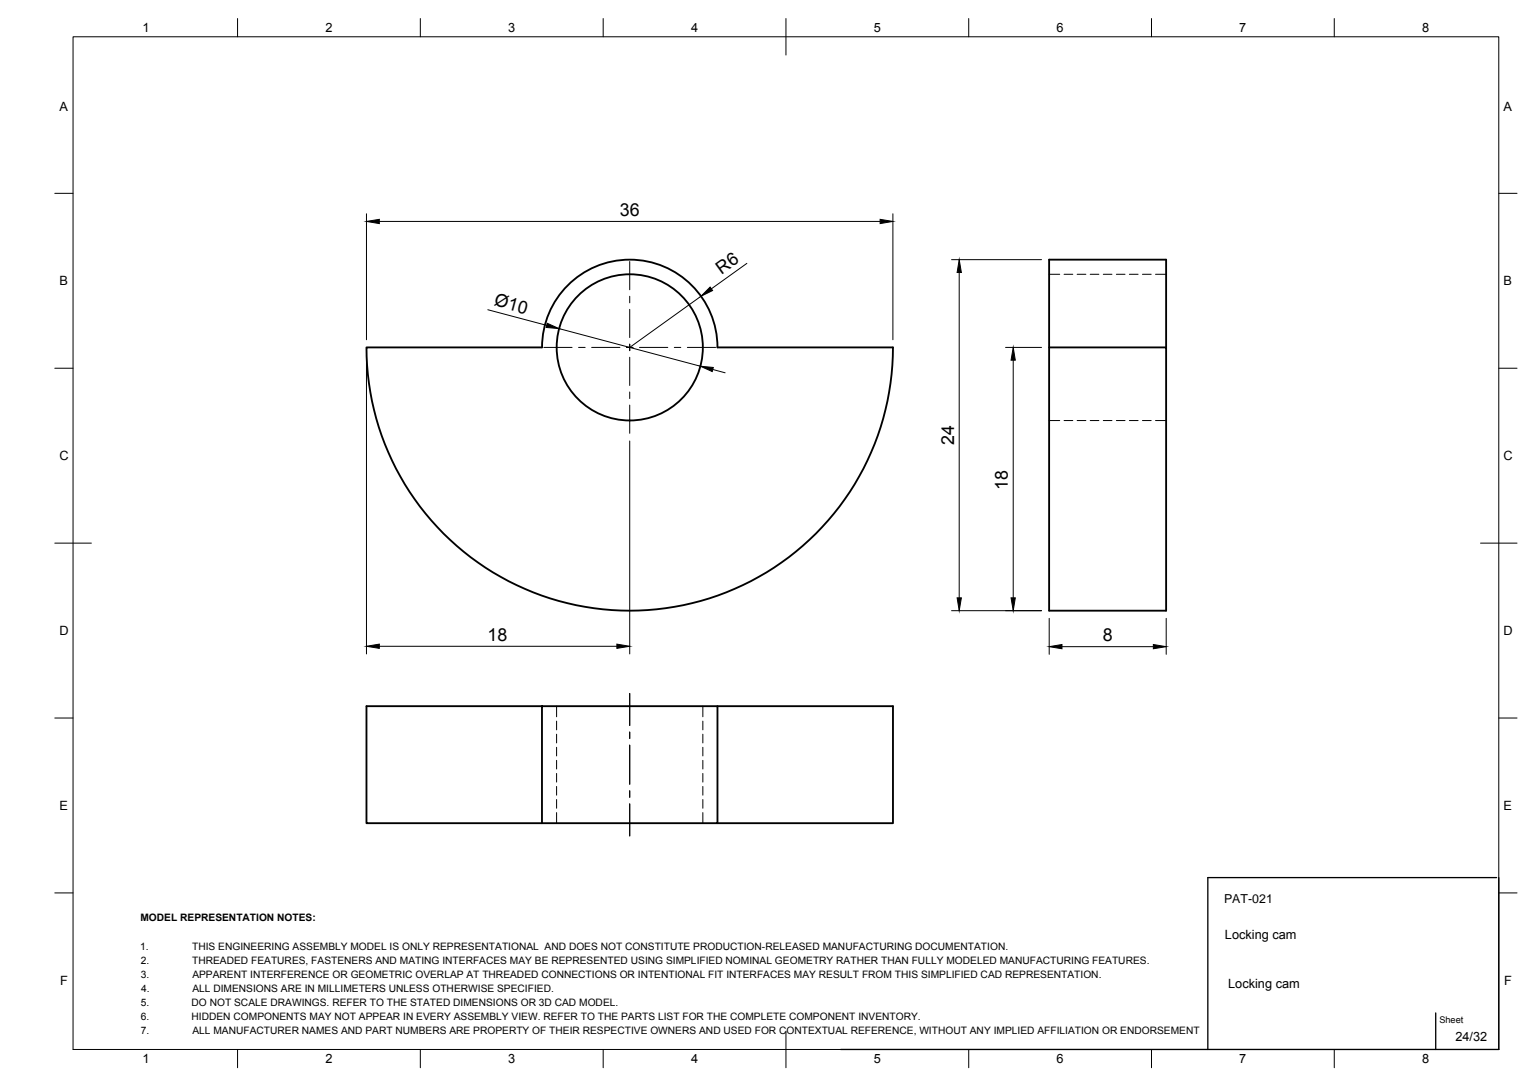
ISO-10303-21;
HEADER;
/* Generated by software containing ST-Developer
 * from STEP Tools, Inc. (www.steptools.com) 
 */

FILE_DESCRIPTION(
/* description */ ('Chain-less indexing wheel (Geneva) drive'),
/* implementation_level */ '2;1');

FILE_NAME(
/* name */ 'Locking cam.step',
/* time_stamp */ '2026-10-28T03:25:22-07:00',
/* author */ (''),
/* organization */ (''),
/* preprocessor_version */ 'ST-DEVELOPER v20.2',
/* originating_system */ 'Autodesk Translation Framework v15.17.0.0',
/* authorisation */ '');

FILE_SCHEMA (('AUTOMOTIVE_DESIGN { 1 0 10303 214 3 1 1 }'));
ENDSEC;

DATA;
#10=MECHANICAL_DESIGN_GEOMETRIC_PRESENTATION_REPRESENTATION('',(#327),#10957);
#269=SHAPE_REPRESENTATION_RELATIONSHIP('SRR','None',#11084,#294);
#294=ADVANCED_BREP_SHAPE_REPRESENTATION('',(#359),#10947);
#327=STYLED_ITEM('',(#11280),#359);
#359=MANIFOLD_SOLID_BREP('Body1',#5724);
#447=FACE_BOUND('',#1284,.T.);
#448=FACE_BOUND('',#1289,.T.);
#579=PLANE('',#6491);
#580=PLANE('',#6493);
#581=PLANE('',#6494);
#582=PLANE('',#6497);
#868=FACE_OUTER_BOUND('',#1281,.T.);
#869=FACE_OUTER_BOUND('',#1282,.T.);
#870=FACE_OUTER_BOUND('',#1283,.T.);
#871=FACE_OUTER_BOUND('',#1285,.T.);
#872=FACE_OUTER_BOUND('',#1286,.T.);
#873=FACE_OUTER_BOUND('',#1287,.T.);
#874=FACE_OUTER_BOUND('',#1288,.T.);
#1281=EDGE_LOOP('',(#4677,#4678,#4679,#4680));
#1282=EDGE_LOOP('',(#4681,#4682,#4683,#4684));
#1283=EDGE_LOOP('',(#4685,#4686,#4687,#4688));
#1284=EDGE_LOOP('',(#4689));
#1285=EDGE_LOOP('',(#4690,#4691,#4692,#4693));
#1286=EDGE_LOOP('',(#4694,#4695,#4696,#4697));
#1287=EDGE_LOOP('',(#4698,#4699,#4700,#4701));
#1288=EDGE_LOOP('',(#4702,#4703,#4704,#4705));
#1289=EDGE_LOOP('',(#4706));
#1625=LINE('',#10145,#1999);
#1626=LINE('',#10150,#2000);
#1627=LINE('',#10154,#2001);
#1628=LINE('',#10158,#2002);
#1629=LINE('',#10161,#2003);
#1630=LINE('',#10164,#2004);
#1631=LINE('',#10165,#2005);
#1632=LINE('',#10168,#2006);
#1633=LINE('',#10169,#2007);
#1999=VECTOR('',#7905,0.5);
#2000=VECTOR('',#7910,1.);
#2001=VECTOR('',#7913,1.);
#2002=VECTOR('',#7918,1.);
#2003=VECTOR('',#7921,1.);
#2004=VECTOR('',#7924,1.);
#2005=VECTOR('',#7925,1.);
#2006=VECTOR('',#7928,1.);
#2007=VECTOR('',#7929,1.);
#2404=CIRCLE('',#6486,0.5);
#2405=CIRCLE('',#6487,0.5);
#2406=CIRCLE('',#6489,0.6);
#2407=CIRCLE('',#6490,0.6);
#2408=CIRCLE('',#6492,1.8);
#2409=CIRCLE('',#6496,1.8);
#2812=VERTEX_POINT('',#10142);
#2813=VERTEX_POINT('',#10144);
#2814=VERTEX_POINT('',#10148);
#2815=VERTEX_POINT('',#10149);
#2816=VERTEX_POINT('',#10151);
#2817=VERTEX_POINT('',#10153);
#2818=VERTEX_POINT('',#10157);
#2819=VERTEX_POINT('',#10159);
#2820=VERTEX_POINT('',#10163);
#2821=VERTEX_POINT('',#10167);
#3464=EDGE_CURVE('',#2812,#2812,#2404,.T.);
#3465=EDGE_CURVE('',#2812,#2813,#1625,.T.);
#3466=EDGE_CURVE('',#2813,#2813,#2405,.T.);
#3467=EDGE_CURVE('',#2814,#2815,#1626,.T.);
#3468=EDGE_CURVE('',#2816,#2814,#2406,.T.);
#3469=EDGE_CURVE('',#2817,#2816,#1627,.T.);
#3470=EDGE_CURVE('',#2817,#2815,#2407,.T.);
#3471=EDGE_CURVE('',#2817,#2818,#1628,.T.);
#3472=EDGE_CURVE('',#2819,#2818,#2408,.T.);
#3473=EDGE_CURVE('',#2819,#2815,#1629,.T.);
#3474=EDGE_CURVE('',#2820,#2816,#1630,.T.);
#3475=EDGE_CURVE('',#2818,#2820,#1631,.T.);
#3476=EDGE_CURVE('',#2821,#2819,#1632,.T.);
#3477=EDGE_CURVE('',#2814,#2821,#1633,.T.);
#3478=EDGE_CURVE('',#2821,#2820,#2409,.T.);
#4677=ORIENTED_EDGE('',*,*,#3464,.F.);
#4678=ORIENTED_EDGE('',*,*,#3465,.T.);
#4679=ORIENTED_EDGE('',*,*,#3466,.F.);
#4680=ORIENTED_EDGE('',*,*,#3465,.F.);
#4681=ORIENTED_EDGE('',*,*,#3467,.F.);
#4682=ORIENTED_EDGE('',*,*,#3468,.F.);
#4683=ORIENTED_EDGE('',*,*,#3469,.F.);
#4684=ORIENTED_EDGE('',*,*,#3470,.T.);
#4685=ORIENTED_EDGE('',*,*,#3471,.T.);
#4686=ORIENTED_EDGE('',*,*,#3472,.F.);
#4687=ORIENTED_EDGE('',*,*,#3473,.T.);
#4688=ORIENTED_EDGE('',*,*,#3470,.F.);
#4689=ORIENTED_EDGE('',*,*,#3464,.T.);
#4690=ORIENTED_EDGE('',*,*,#3469,.T.);
#4691=ORIENTED_EDGE('',*,*,#3474,.F.);
#4692=ORIENTED_EDGE('',*,*,#3475,.F.);
#4693=ORIENTED_EDGE('',*,*,#3471,.F.);
#4694=ORIENTED_EDGE('',*,*,#3467,.T.);
#4695=ORIENTED_EDGE('',*,*,#3473,.F.);
#4696=ORIENTED_EDGE('',*,*,#3476,.F.);
#4697=ORIENTED_EDGE('',*,*,#3477,.F.);
#4698=ORIENTED_EDGE('',*,*,#3476,.T.);
#4699=ORIENTED_EDGE('',*,*,#3472,.T.);
#4700=ORIENTED_EDGE('',*,*,#3475,.T.);
#4701=ORIENTED_EDGE('',*,*,#3478,.F.);
#4702=ORIENTED_EDGE('',*,*,#3477,.T.);
#4703=ORIENTED_EDGE('',*,*,#3478,.T.);
#4704=ORIENTED_EDGE('',*,*,#3474,.T.);
#4705=ORIENTED_EDGE('',*,*,#3468,.T.);
#4706=ORIENTED_EDGE('',*,*,#3466,.T.);
#5326=CYLINDRICAL_SURFACE('',#6485,0.5);
#5327=CYLINDRICAL_SURFACE('',#6488,0.6);
#5328=CYLINDRICAL_SURFACE('',#6495,1.8);
#5582=ADVANCED_FACE('',(#868),#5326,.F.);
#5583=ADVANCED_FACE('',(#869),#5327,.T.);
#5584=ADVANCED_FACE('',(#870,#447),#579,.F.);
#5585=ADVANCED_FACE('',(#871),#580,.F.);
#5586=ADVANCED_FACE('',(#872),#581,.F.);
#5587=ADVANCED_FACE('',(#873),#5328,.T.);
#5588=ADVANCED_FACE('',(#874,#448),#582,.T.);
#5724=CLOSED_SHELL('',(#5582,#5583,#5584,#5585,#5586,#5587,#5588));
#6484=AXIS2_PLACEMENT_3D('',#10140,#7899,#7900);
#6485=AXIS2_PLACEMENT_3D('',#10141,#7901,#7902);
#6486=AXIS2_PLACEMENT_3D('',#10143,#7903,#7904);
#6487=AXIS2_PLACEMENT_3D('',#10146,#7906,#7907);
#6488=AXIS2_PLACEMENT_3D('',#10147,#7908,#7909);
#6489=AXIS2_PLACEMENT_3D('',#10152,#7911,#7912);
#6490=AXIS2_PLACEMENT_3D('',#10155,#7914,#7915);
#6491=AXIS2_PLACEMENT_3D('',#10156,#7916,#7917);
#6492=AXIS2_PLACEMENT_3D('',#10160,#7919,#7920);
#6493=AXIS2_PLACEMENT_3D('',#10162,#7922,#7923);
#6494=AXIS2_PLACEMENT_3D('',#10166,#7926,#7927);
#6495=AXIS2_PLACEMENT_3D('',#10170,#7930,#7931);
#6496=AXIS2_PLACEMENT_3D('',#10171,#7932,#7933);
#6497=AXIS2_PLACEMENT_3D('',#10172,#7934,#7935);
#7899=DIRECTION('axis',(0.,0.,1.));
#7900=DIRECTION('refdir',(1.,0.,0.));
#7901=DIRECTION('center_axis',(0.,0.,1.));
#7902=DIRECTION('ref_axis',(1.,0.,0.));
#7903=DIRECTION('center_axis',(0.,0.,1.));
#7904=DIRECTION('ref_axis',(1.,0.,0.));
#7905=DIRECTION('',(0.,0.,1.));
#7906=DIRECTION('center_axis',(0.,0.,-1.));
#7907=DIRECTION('ref_axis',(1.,0.,0.));
#7908=DIRECTION('center_axis',(0.,0.,1.));
#7909=DIRECTION('ref_axis',(1.,0.,0.));
#7910=DIRECTION('',(0.,0.,-1.));
#7911=DIRECTION('center_axis',(0.,0.,1.));
#7912=DIRECTION('ref_axis',(1.,0.,0.));
#7913=DIRECTION('',(0.,0.,1.));
#7914=DIRECTION('center_axis',(0.,0.,1.));
#7915=DIRECTION('ref_axis',(1.,0.,0.));
#7916=DIRECTION('center_axis',(0.,0.,1.));
#7917=DIRECTION('ref_axis',(1.,0.,0.));
#7918=DIRECTION('',(0.,-1.,0.));
#7919=DIRECTION('center_axis',(0.,0.,1.));
#7920=DIRECTION('ref_axis',(1.,0.,0.));
#7921=DIRECTION('',(0.,-1.,0.));
#7922=DIRECTION('center_axis',(-1.,0.,0.));
#7923=DIRECTION('ref_axis',(0.,-1.,0.));
#7924=DIRECTION('',(0.,1.,0.));
#7925=DIRECTION('',(0.,0.,1.));
#7926=DIRECTION('center_axis',(-1.,0.,0.));
#7927=DIRECTION('ref_axis',(0.,-1.,0.));
#7928=DIRECTION('',(0.,0.,-1.));
#7929=DIRECTION('',(0.,1.,0.));
#7930=DIRECTION('center_axis',(0.,0.,1.));
#7931=DIRECTION('ref_axis',(-1.,1.22464679914735E-16,0.));
#7932=DIRECTION('center_axis',(0.,0.,1.));
#7933=DIRECTION('ref_axis',(1.,0.,0.));
#7934=DIRECTION('center_axis',(0.,0.,1.));
#7935=DIRECTION('ref_axis',(1.,0.,0.));
#10140=CARTESIAN_POINT('',(0.,0.,0.));
#10141=CARTESIAN_POINT('Origin',(0.,0.,5.9));
#10142=CARTESIAN_POINT('',(-0.5,-6.12323399573677E-17,6.));
#10143=CARTESIAN_POINT('Origin',(0.,0.,6.));
#10144=CARTESIAN_POINT('',(-0.5,6.12323399573677E-17,6.8));
#10145=CARTESIAN_POINT('',(-0.5,-6.12323399573677E-17,5.9));
#10146=CARTESIAN_POINT('Origin',(0.,0.,6.8));
#10147=CARTESIAN_POINT('Origin',(0.,0.,6.));
#10148=CARTESIAN_POINT('',(0.,0.6,6.8));
#10149=CARTESIAN_POINT('',(0.,0.6,6.));
#10150=CARTESIAN_POINT('',(0.,0.6,6.));
#10151=CARTESIAN_POINT('',(0.,-0.6,6.8));
#10152=CARTESIAN_POINT('Origin',(0.,0.,6.8));
#10153=CARTESIAN_POINT('',(0.,-0.6,6.));
#10154=CARTESIAN_POINT('',(0.,-0.6,6.));
#10155=CARTESIAN_POINT('Origin',(0.,0.,6.));
#10156=CARTESIAN_POINT('Origin',(0.,0.,6.));
#10157=CARTESIAN_POINT('',(0.,-1.8,6.));
#10158=CARTESIAN_POINT('',(0.,0.95,6.));
#10159=CARTESIAN_POINT('',(0.,1.8,6.));
#10160=CARTESIAN_POINT('Origin',(0.,0.,6.));
#10161=CARTESIAN_POINT('',(0.,0.95,6.));
#10162=CARTESIAN_POINT('Origin',(0.,1.9,5.9));
#10163=CARTESIAN_POINT('',(0.,-1.8,6.8));
#10164=CARTESIAN_POINT('',(0.,0.95,6.8));
#10165=CARTESIAN_POINT('',(0.,-1.8,6.));
#10166=CARTESIAN_POINT('Origin',(0.,1.9,5.9));
#10167=CARTESIAN_POINT('',(0.,1.8,6.8));
#10168=CARTESIAN_POINT('',(0.,1.8,6.));
#10169=CARTESIAN_POINT('',(0.,0.95,6.8));
#10170=CARTESIAN_POINT('Origin',(0.,0.,6.));
#10171=CARTESIAN_POINT('Origin',(0.,0.,6.8));
#10172=CARTESIAN_POINT('Origin',(0.,0.,6.8));
#10916=UNCERTAINTY_MEASURE_WITH_UNIT(LENGTH_MEASURE(0.001),#10958,
'DISTANCE_ACCURACY_VALUE',
'Maximum model space distance between geometric entities at asserted c
onnectivities');
#10926=UNCERTAINTY_MEASURE_WITH_UNIT(LENGTH_MEASURE(0.001),#10958,
'DISTANCE_ACCURACY_VALUE',
'Maximum model space distance between geometric entities at asserted c
onnectivities');
#10947=(
GEOMETRIC_REPRESENTATION_CONTEXT(3)
GLOBAL_UNCERTAINTY_ASSIGNED_CONTEXT((#10916))
GLOBAL_UNIT_ASSIGNED_CONTEXT((#10958,#10960,#10961))
REPRESENTATION_CONTEXT('','3D')
);
#10957=(
GEOMETRIC_REPRESENTATION_CONTEXT(3)
GLOBAL_UNCERTAINTY_ASSIGNED_CONTEXT((#10926))
GLOBAL_UNIT_ASSIGNED_CONTEXT((#10958,#10960,#10961))
REPRESENTATION_CONTEXT('','3D')
);
#10958=(
LENGTH_UNIT()
NAMED_UNIT(*)
SI_UNIT(.CENTI.,.METRE.)
);
#10960=(
NAMED_UNIT(*)
PLANE_ANGLE_UNIT()
SI_UNIT($,.RADIAN.)
);
#10961=(
NAMED_UNIT(*)
SI_UNIT($,.STERADIAN.)
SOLID_ANGLE_UNIT()
);
#10982=SHAPE_DEFINITION_REPRESENTATION(#11017,#11084);
#11017=PRODUCT_DEFINITION_SHAPE('',$,#11115);
#11084=SHAPE_REPRESENTATION('',(#6484),#10947);
#11094=PRODUCT_DEFINITION_CONTEXT('part definition',#11186,'design');
#11115=PRODUCT_DEFINITION('Locking cam','Locking cam',#11145,#11094);
#11145=PRODUCT_DEFINITION_FORMATION('',$,#11208);
#11186=APPLICATION_CONTEXT(
'Core Data for Automotive Mechanical Design Process');
#11187=PRODUCT_CONTEXT('part definition',#11186,'mechanical');
#11208=PRODUCT('Locking cam','Locking cam','Locking cam',(#11187));
#11274=COLOUR_RGB('Sky Blue',0.24,0.69,0.87);
#11275=FILL_AREA_STYLE_COLOUR('',#11274);
#11276=FILL_AREA_STYLE('',(#11275));
#11277=SURFACE_STYLE_FILL_AREA(#11276);
#11278=SURFACE_SIDE_STYLE('',(#11277));
#11279=SURFACE_STYLE_USAGE(.BOTH.,#11278);
#11280=PRESENTATION_STYLE_ASSIGNMENT((#11279));
ENDSEC;
END-ISO-10303-21;
